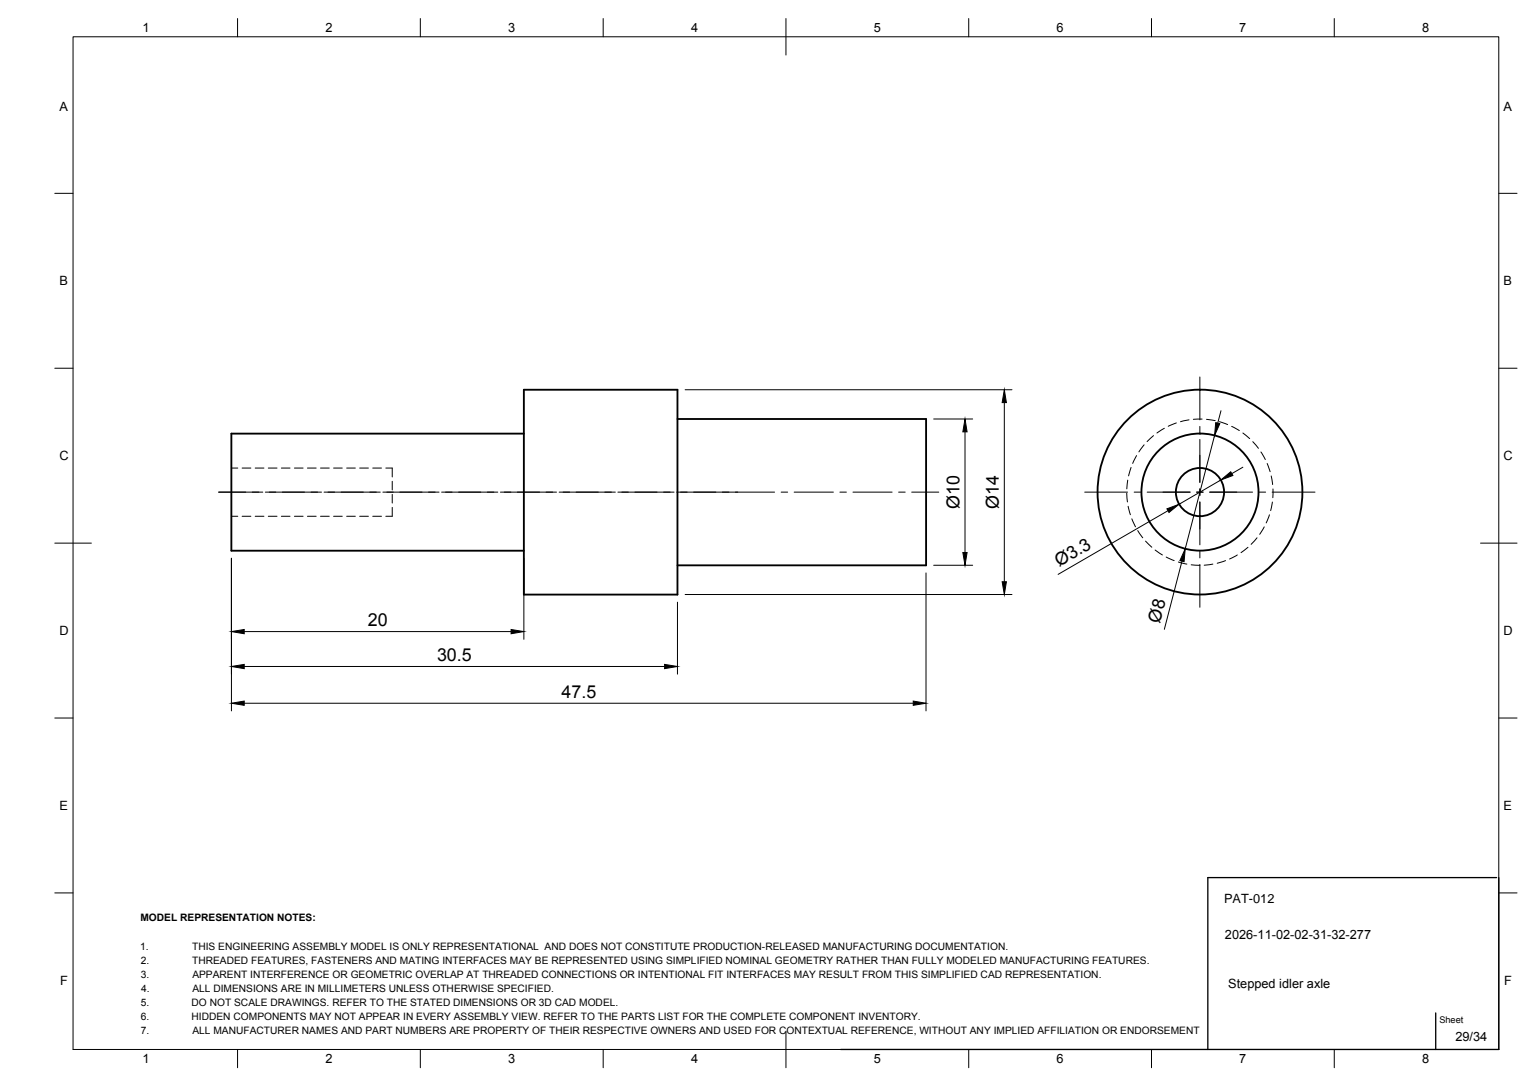
ISO-10303-21;
HEADER;
/* Generated by software containing ST-Developer
 * from STEP Tools, Inc. (www.steptools.com) 
 */

FILE_DESCRIPTION(
/* description */ ('Belt tensioner idler arm'),
/* implementation_level */ '2;1');

FILE_NAME(
/* name */ 'Stepped idler axle.step',
/* time_stamp */ '2026-10-28T03:22:15-07:00',
/* author */ (''),
/* organization */ (''),
/* preprocessor_version */ 'ST-DEVELOPER v20.2',
/* originating_system */ 'Autodesk Translation Framework v15.17.0.0',
/* authorisation */ '');

FILE_SCHEMA (('AUTOMOTIVE_DESIGN { 1 0 10303 214 3 1 1 }'));
ENDSEC;

DATA;
#10=MECHANICAL_DESIGN_GEOMETRIC_PRESENTATION_REPRESENTATION('',(#479),#12779);
#403=SHAPE_REPRESENTATION_RELATIONSHIP('SRR','None',#12952,#437);
#437=ADVANCED_BREP_SHAPE_REPRESENTATION('',(#518),#12769);
#479=STYLED_ITEM('',(#13184),#518);
#518=MANIFOLD_SOLID_BREP('Body1',#6216);
#637=FACE_BOUND('',#1571,.T.);
#638=FACE_BOUND('',#1573,.T.);
#639=FACE_BOUND('',#1577,.T.);
#793=PLANE('',#7153);
#794=PLANE('',#7157);
#795=PLANE('',#7158);
#796=PLANE('',#7165);
#797=PLANE('',#7166);
#1090=FACE_OUTER_BOUND('',#1567,.T.);
#1091=FACE_OUTER_BOUND('',#1568,.T.);
#1092=FACE_OUTER_BOUND('',#1569,.T.);
#1093=FACE_OUTER_BOUND('',#1570,.T.);
#1094=FACE_OUTER_BOUND('',#1572,.T.);
#1095=FACE_OUTER_BOUND('',#1574,.T.);
#1096=FACE_OUTER_BOUND('',#1575,.T.);
#1097=FACE_OUTER_BOUND('',#1576,.T.);
#1098=FACE_OUTER_BOUND('',#1578,.T.);
#1567=EDGE_LOOP('',(#5132,#5133,#5134,#5135));
#1568=EDGE_LOOP('',(#5136));
#1569=EDGE_LOOP('',(#5137,#5138,#5139,#5140));
#1570=EDGE_LOOP('',(#5141));
#1571=EDGE_LOOP('',(#5142));
#1572=EDGE_LOOP('',(#5143));
#1573=EDGE_LOOP('',(#5144));
#1574=EDGE_LOOP('',(#5145,#5146,#5147,#5148));
#1575=EDGE_LOOP('',(#5149,#5150,#5151,#5152));
#1576=EDGE_LOOP('',(#5153));
#1577=EDGE_LOOP('',(#5154));
#1578=EDGE_LOOP('',(#5155));
#1946=LINE('',#11766,#2295);
#1947=LINE('',#11773,#2296);
#1948=LINE('',#11784,#2297);
#1949=LINE('',#11787,#2298);
#2295=VECTOR('',#8772,0.164999999999999);
#2296=VECTOR('',#8781,0.4);
#2297=VECTOR('',#8796,0.699999999999999);
#2298=VECTOR('',#8799,0.5);
#2641=CIRCLE('',#7151,0.164999999999999);
#2642=CIRCLE('',#7152,0.164999999999999);
#2643=CIRCLE('',#7155,0.4);
#2644=CIRCLE('',#7156,0.4);
#2645=CIRCLE('',#7159,0.699999999999999);
#2646=CIRCLE('',#7160,0.5);
#2647=CIRCLE('',#7162,0.699999999999999);
#2648=CIRCLE('',#7164,0.5);
#3119=VERTEX_POINT('',#11763);
#3120=VERTEX_POINT('',#11765);
#3121=VERTEX_POINT('',#11770);
#3122=VERTEX_POINT('',#11772);
#3123=VERTEX_POINT('',#11777);
#3124=VERTEX_POINT('',#11779);
#3125=VERTEX_POINT('',#11782);
#3126=VERTEX_POINT('',#11786);
#3821=EDGE_CURVE('',#3119,#3119,#2641,.T.);
#3822=EDGE_CURVE('',#3119,#3120,#1946,.T.);
#3823=EDGE_CURVE('',#3120,#3120,#2642,.T.);
#3824=EDGE_CURVE('',#3121,#3121,#2643,.T.);
#3825=EDGE_CURVE('',#3121,#3122,#1947,.T.);
#3826=EDGE_CURVE('',#3122,#3122,#2644,.T.);
#3827=EDGE_CURVE('',#3123,#3123,#2645,.T.);
#3828=EDGE_CURVE('',#3124,#3124,#2646,.T.);
#3829=EDGE_CURVE('',#3125,#3125,#2647,.T.);
#3830=EDGE_CURVE('',#3125,#3123,#1948,.T.);
#3831=EDGE_CURVE('',#3124,#3126,#1949,.T.);
#3832=EDGE_CURVE('',#3126,#3126,#2648,.T.);
#5132=ORIENTED_EDGE('',*,*,#3821,.F.);
#5133=ORIENTED_EDGE('',*,*,#3822,.T.);
#5134=ORIENTED_EDGE('',*,*,#3823,.F.);
#5135=ORIENTED_EDGE('',*,*,#3822,.F.);
#5136=ORIENTED_EDGE('',*,*,#3821,.T.);
#5137=ORIENTED_EDGE('',*,*,#3824,.F.);
#5138=ORIENTED_EDGE('',*,*,#3825,.T.);
#5139=ORIENTED_EDGE('',*,*,#3826,.F.);
#5140=ORIENTED_EDGE('',*,*,#3825,.F.);
#5141=ORIENTED_EDGE('',*,*,#3824,.T.);
#5142=ORIENTED_EDGE('',*,*,#3823,.T.);
#5143=ORIENTED_EDGE('',*,*,#3827,.F.);
#5144=ORIENTED_EDGE('',*,*,#3828,.F.);
#5145=ORIENTED_EDGE('',*,*,#3829,.F.);
#5146=ORIENTED_EDGE('',*,*,#3830,.T.);
#5147=ORIENTED_EDGE('',*,*,#3827,.T.);
#5148=ORIENTED_EDGE('',*,*,#3830,.F.);
#5149=ORIENTED_EDGE('',*,*,#3828,.T.);
#5150=ORIENTED_EDGE('',*,*,#3831,.T.);
#5151=ORIENTED_EDGE('',*,*,#3832,.T.);
#5152=ORIENTED_EDGE('',*,*,#3831,.F.);
#5153=ORIENTED_EDGE('',*,*,#3829,.T.);
#5154=ORIENTED_EDGE('',*,*,#3826,.T.);
#5155=ORIENTED_EDGE('',*,*,#3832,.F.);
#5748=CYLINDRICAL_SURFACE('',#7150,0.164999999999999);
#5749=CYLINDRICAL_SURFACE('',#7154,0.4);
#5750=CYLINDRICAL_SURFACE('',#7161,0.699999999999999);
#5751=CYLINDRICAL_SURFACE('',#7163,0.5);
#6067=ADVANCED_FACE('',(#1090),#5748,.F.);
#6068=ADVANCED_FACE('',(#1091),#793,.T.);
#6069=ADVANCED_FACE('',(#1092),#5749,.T.);
#6070=ADVANCED_FACE('',(#1093,#637),#794,.T.);
#6071=ADVANCED_FACE('',(#1094,#638),#795,.F.);
#6072=ADVANCED_FACE('',(#1095),#5750,.T.);
#6073=ADVANCED_FACE('',(#1096),#5751,.T.);
#6074=ADVANCED_FACE('',(#1097,#639),#796,.T.);
#6075=ADVANCED_FACE('',(#1098),#797,.F.);
#6216=CLOSED_SHELL('',(#6067,#6068,#6069,#6070,#6071,#6072,#6073,#6074,
#6075));
#7149=AXIS2_PLACEMENT_3D('',#11761,#8766,#8767);
#7150=AXIS2_PLACEMENT_3D('',#11762,#8768,#8769);
#7151=AXIS2_PLACEMENT_3D('',#11764,#8770,#8771);
#7152=AXIS2_PLACEMENT_3D('',#11767,#8773,#8774);
#7153=AXIS2_PLACEMENT_3D('',#11768,#8775,#8776);
#7154=AXIS2_PLACEMENT_3D('',#11769,#8777,#8778);
#7155=AXIS2_PLACEMENT_3D('',#11771,#8779,#8780);
#7156=AXIS2_PLACEMENT_3D('',#11774,#8782,#8783);
#7157=AXIS2_PLACEMENT_3D('',#11775,#8784,#8785);
#7158=AXIS2_PLACEMENT_3D('',#11776,#8786,#8787);
#7159=AXIS2_PLACEMENT_3D('',#11778,#8788,#8789);
#7160=AXIS2_PLACEMENT_3D('',#11780,#8790,#8791);
#7161=AXIS2_PLACEMENT_3D('',#11781,#8792,#8793);
#7162=AXIS2_PLACEMENT_3D('',#11783,#8794,#8795);
#7163=AXIS2_PLACEMENT_3D('',#11785,#8797,#8798);
#7164=AXIS2_PLACEMENT_3D('',#11788,#8800,#8801);
#7165=AXIS2_PLACEMENT_3D('',#11789,#8802,#8803);
#7166=AXIS2_PLACEMENT_3D('',#11790,#8804,#8805);
#8766=DIRECTION('axis',(0.,0.,1.));
#8767=DIRECTION('refdir',(1.,0.,0.));
#8768=DIRECTION('center_axis',(0.,0.,1.));
#8769=DIRECTION('ref_axis',(1.,0.,0.));
#8770=DIRECTION('center_axis',(0.,0.,1.));
#8771=DIRECTION('ref_axis',(1.,0.,0.));
#8772=DIRECTION('',(0.,0.,1.));
#8773=DIRECTION('center_axis',(0.,0.,-1.));
#8774=DIRECTION('ref_axis',(1.,0.,0.));
#8775=DIRECTION('center_axis',(0.,0.,1.));
#8776=DIRECTION('ref_axis',(1.,0.,0.));
#8777=DIRECTION('center_axis',(0.,0.,1.));
#8778=DIRECTION('ref_axis',(1.,0.,0.));
#8779=DIRECTION('center_axis',(0.,0.,1.));
#8780=DIRECTION('ref_axis',(1.,0.,0.));
#8781=DIRECTION('',(0.,0.,-1.));
#8782=DIRECTION('center_axis',(0.,0.,-1.));
#8783=DIRECTION('ref_axis',(1.,0.,0.));
#8784=DIRECTION('center_axis',(0.,0.,1.));
#8785=DIRECTION('ref_axis',(1.,0.,0.));
#8786=DIRECTION('center_axis',(0.,0.,1.));
#8787=DIRECTION('ref_axis',(1.,0.,0.));
#8788=DIRECTION('center_axis',(0.,0.,1.));
#8789=DIRECTION('ref_axis',(1.,0.,0.));
#8790=DIRECTION('center_axis',(0.,0.,-1.));
#8791=DIRECTION('ref_axis',(1.,0.,0.));
#8792=DIRECTION('center_axis',(0.,0.,1.));
#8793=DIRECTION('ref_axis',(1.,0.,0.));
#8794=DIRECTION('center_axis',(0.,0.,1.));
#8795=DIRECTION('ref_axis',(1.,0.,0.));
#8796=DIRECTION('',(0.,0.,-1.));
#8797=DIRECTION('center_axis',(0.,0.,1.));
#8798=DIRECTION('ref_axis',(1.,0.,0.));
#8799=DIRECTION('',(0.,0.,-1.));
#8800=DIRECTION('center_axis',(0.,0.,1.));
#8801=DIRECTION('ref_axis',(1.,0.,0.));
#8802=DIRECTION('center_axis',(0.,0.,1.));
#8803=DIRECTION('ref_axis',(1.,0.,0.));
#8804=DIRECTION('center_axis',(0.,0.,1.));
#8805=DIRECTION('ref_axis',(1.,0.,0.));
#11761=CARTESIAN_POINT('',(0.,0.,0.));
#11762=CARTESIAN_POINT('Origin',(9.,0.,7.9));
#11763=CARTESIAN_POINT('',(8.835,-2.02066721859312E-17,7.9));
#11764=CARTESIAN_POINT('Origin',(9.,0.,7.9));
#11765=CARTESIAN_POINT('',(8.835,2.02066721859312E-17,9.));
#11766=CARTESIAN_POINT('',(8.835,-2.02066721859312E-17,7.9));
#11767=CARTESIAN_POINT('Origin',(9.,0.,9.));
#11768=CARTESIAN_POINT('Origin',(9.,0.,7.9));
#11769=CARTESIAN_POINT('Origin',(9.,0.,7.));
#11770=CARTESIAN_POINT('',(8.6,-4.89858719658942E-17,9.));
#11771=CARTESIAN_POINT('Origin',(9.,0.,9.));
#11772=CARTESIAN_POINT('',(8.6,-4.89858719658942E-17,7.));
#11773=CARTESIAN_POINT('',(8.6,-4.89858719658942E-17,7.));
#11774=CARTESIAN_POINT('Origin',(9.,0.,7.));
#11775=CARTESIAN_POINT('Origin',(9.,0.,9.));
#11776=CARTESIAN_POINT('Origin',(9.,0.,5.95));
#11777=CARTESIAN_POINT('',(8.3,-8.57252759403146E-17,5.95));
#11778=CARTESIAN_POINT('Origin',(9.,0.,5.95));
#11779=CARTESIAN_POINT('',(8.5,6.12323399573677E-17,5.95));
#11780=CARTESIAN_POINT('Origin',(9.,0.,5.95));
#11781=CARTESIAN_POINT('Origin',(9.,0.,5.95));
#11782=CARTESIAN_POINT('',(8.3,-8.57252759403146E-17,7.));
#11783=CARTESIAN_POINT('Origin',(9.,0.,7.));
#11784=CARTESIAN_POINT('',(8.3,-8.57252759403146E-17,5.95));
#11785=CARTESIAN_POINT('Origin',(9.,0.,4.25));
#11786=CARTESIAN_POINT('',(8.5,-6.12323399573677E-17,4.25));
#11787=CARTESIAN_POINT('',(8.5,-6.12323399573677E-17,4.25));
#11788=CARTESIAN_POINT('Origin',(9.,0.,4.25));
#11789=CARTESIAN_POINT('Origin',(9.,0.,7.));
#11790=CARTESIAN_POINT('Origin',(9.,0.,4.25));
#12729=UNCERTAINTY_MEASURE_WITH_UNIT(LENGTH_MEASURE(0.001),#12780,
'DISTANCE_ACCURACY_VALUE',
'Maximum model space distance between geometric entities at asserted c
onnectivities');
#12739=UNCERTAINTY_MEASURE_WITH_UNIT(LENGTH_MEASURE(0.001),#12780,
'DISTANCE_ACCURACY_VALUE',
'Maximum model space distance between geometric entities at asserted c
onnectivities');
#12769=(
GEOMETRIC_REPRESENTATION_CONTEXT(3)
GLOBAL_UNCERTAINTY_ASSIGNED_CONTEXT((#12729))
GLOBAL_UNIT_ASSIGNED_CONTEXT((#12780,#12782,#12783))
REPRESENTATION_CONTEXT('','3D')
);
#12779=(
GEOMETRIC_REPRESENTATION_CONTEXT(3)
GLOBAL_UNCERTAINTY_ASSIGNED_CONTEXT((#12739))
GLOBAL_UNIT_ASSIGNED_CONTEXT((#12780,#12782,#12783))
REPRESENTATION_CONTEXT('','3D')
);
#12780=(
LENGTH_UNIT()
NAMED_UNIT(*)
SI_UNIT(.CENTI.,.METRE.)
);
#12782=(
NAMED_UNIT(*)
PLANE_ANGLE_UNIT()
SI_UNIT($,.RADIAN.)
);
#12783=(
NAMED_UNIT(*)
SI_UNIT($,.STERADIAN.)
SOLID_ANGLE_UNIT()
);
#12813=SHAPE_DEFINITION_REPRESENTATION(#12881,#12952);
#12881=PRODUCT_DEFINITION_SHAPE('',$,#12992);
#12952=SHAPE_REPRESENTATION('',(#7149),#12769);
#12962=PRODUCT_DEFINITION_CONTEXT('part definition',#13081,'design');
#12992=PRODUCT_DEFINITION('Stepped idler axle','Stepped idler axle',#13031,
#12962);
#13031=PRODUCT_DEFINITION_FORMATION('',$,#13112);
#13081=APPLICATION_CONTEXT(
'Core Data for Automotive Mechanical Design Process');
#13082=PRODUCT_CONTEXT('part definition',#13081,'mechanical');
#13112=PRODUCT('Stepped idler axle','Stepped idler axle',
'Stepped idler axle',(#13082));
#13178=COLOUR_RGB('Grey',0.48,0.52,0.57);
#13179=FILL_AREA_STYLE_COLOUR('',#13178);
#13180=FILL_AREA_STYLE('',(#13179));
#13181=SURFACE_STYLE_FILL_AREA(#13180);
#13182=SURFACE_SIDE_STYLE('',(#13181));
#13183=SURFACE_STYLE_USAGE(.BOTH.,#13182);
#13184=PRESENTATION_STYLE_ASSIGNMENT((#13183));
ENDSEC;
END-ISO-10303-21;
